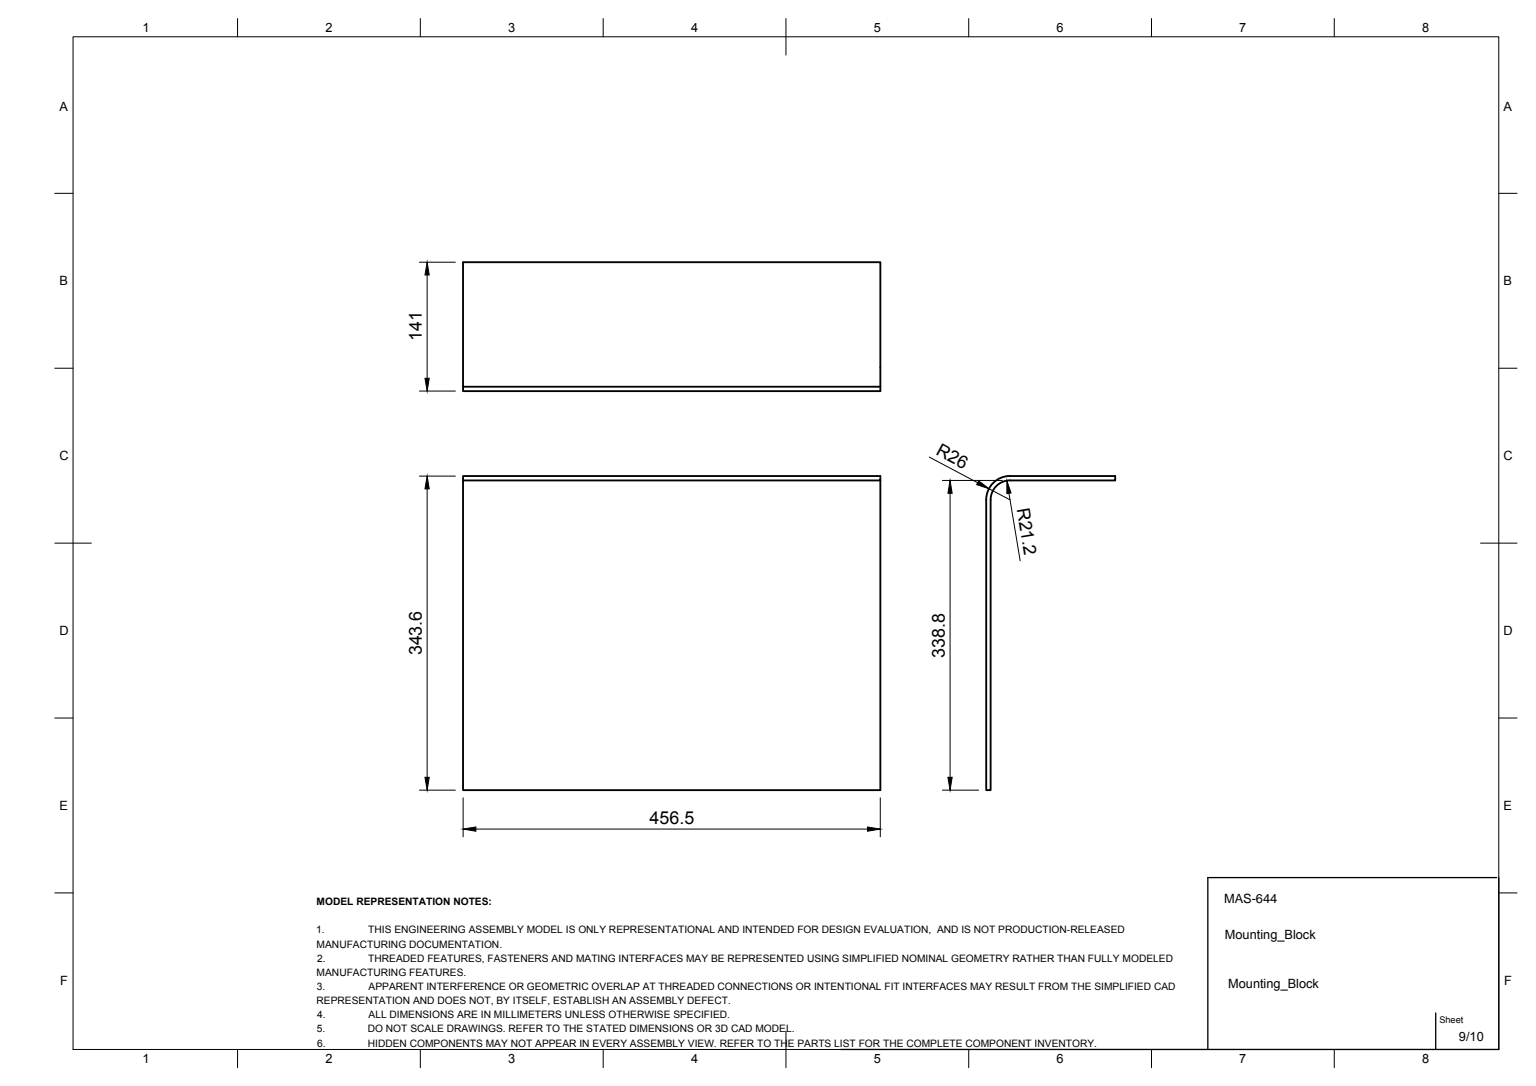
ISO-10303-21;
HEADER;
FILE_DESCRIPTION((''),'2;1');
FILE_NAME('Mounting_Block.step','2026-10-09T11:38:21-07:00',(''),(''),'','','');
FILE_SCHEMA (('AUTOMOTIVE_DESIGN { 1 0 10303 214 3 1 1 }'));
ENDSEC;
DATA;
#10=MECHANICAL_DESIGN_GEOMETRIC_PRESENTATION_REPRESENTATION('',(#65),#3619);
#49=SHAPE_REPRESENTATION_RELATIONSHIP('SRR','None',#3657,#57) ;
#57=ADVANCED_BREP_SHAPE_REPRESENTATION('',(#73),#3617) ;
#65=STYLED_ITEM('',(#3700),#73) ;
#73=MANIFOLD_SOLID_BREP('Body1',#2089) ;
#197=PLANE('',#2372) ;
#198=PLANE('',#2375) ;
#199=PLANE('',#2376) ;
#200=PLANE('',#2379) ;
#201=PLANE('',#2380) ;
#202=PLANE('',#2381) ;
#203=PLANE('',#2382) ;
#204=PLANE('',#2384) ;
#205=PLANE('',#2385) ;
#206=PLANE('',#2386) ;
#207=PLANE('',#2388) ;
#208=PLANE('',#2389) ;
#301=FACE_OUTER_BOUND('',#491,.T.) ;
#302=FACE_OUTER_BOUND('',#492,.T.) ;
#303=FACE_OUTER_BOUND('',#493,.T.) ;
#304=FACE_OUTER_BOUND('',#494,.T.) ;
#305=FACE_OUTER_BOUND('',#495,.T.) ;
#306=FACE_OUTER_BOUND('',#496,.T.) ;
#307=FACE_OUTER_BOUND('',#497,.T.) ;
#308=FACE_OUTER_BOUND('',#498,.T.) ;
#309=FACE_OUTER_BOUND('',#499,.T.) ;
#310=FACE_OUTER_BOUND('',#500,.T.) ;
#311=FACE_OUTER_BOUND('',#501,.T.) ;
#312=FACE_OUTER_BOUND('',#502,.T.) ;
#313=FACE_OUTER_BOUND('',#503,.T.) ;
#314=FACE_OUTER_BOUND('',#504,.T.) ;
#491=EDGE_LOOP('',(#1843,#1844,#1845,#1846)) ;
#492=EDGE_LOOP('',(#1847,#1848,#1849,#1850)) ;
#493=EDGE_LOOP('',(#1851,#1852,#1853,#1854)) ;
#494=EDGE_LOOP('',(#1855,#1856,#1857,#1858)) ;
#495=EDGE_LOOP('',(#1859,#1860,#1861,#1862)) ;
#496=EDGE_LOOP('',(#1863,#1864,#1865,#1866)) ;
#497=EDGE_LOOP('',(#1867,#1868,#1869,#1870)) ;
#498=EDGE_LOOP('',(#1871,#1872,#1873,#1874)) ;
#499=EDGE_LOOP('',(#1875,#1876,#1877,#1878)) ;
#500=EDGE_LOOP('',(#1879,#1880,#1881,#1882)) ;
#501=EDGE_LOOP('',(#1883,#1884,#1885,#1886)) ;
#502=EDGE_LOOP('',(#1887,#1888,#1889,#1890)) ;
#503=EDGE_LOOP('',(#1891,#1892,#1893,#1894)) ;
#504=EDGE_LOOP('',(#1895,#1896,#1897,#1898)) ;
#643=LINE('',#3510,#807) ;
#644=LINE('',#3514,#808) ;
#645=LINE('',#3518,#809) ;
#646=LINE('',#3520,#810) ;
#647=LINE('',#3521,#811) ;
#648=LINE('',#3525,#812) ;
#649=LINE('',#3529,#813) ;
#650=LINE('',#3533,#814) ;
#651=LINE('',#3535,#815) ;
#652=LINE('',#3536,#816) ;
#653=LINE('',#3539,#817) ;
#654=LINE('',#3540,#818) ;
#655=LINE('',#3541,#819) ;
#656=LINE('',#3544,#820) ;
#657=LINE('',#3545,#821) ;
#658=LINE('',#3547,#822) ;
#659=LINE('',#3548,#823) ;
#660=LINE('',#3550,#824) ;
#661=LINE('',#3553,#825) ;
#662=LINE('',#3554,#826) ;
#663=LINE('',#3557,#827) ;
#664=LINE('',#3558,#828) ;
#665=LINE('',#3560,#829) ;
#666=LINE('',#3561,#830) ;
#807=VECTOR('',#2927,1000.) ;
#808=VECTOR('',#2930,1000.) ;
#809=VECTOR('',#2935,1000.) ;
#810=VECTOR('',#2936,1000.) ;
#811=VECTOR('',#2937,1000.) ;
#812=VECTOR('',#2940,1000.) ;
#813=VECTOR('',#2943,1000.) ;
#814=VECTOR('',#2948,1000.) ;
#815=VECTOR('',#2949,1000.) ;
#816=VECTOR('',#2950,1000.) ;
#817=VECTOR('',#2953,1000.) ;
#818=VECTOR('',#2954,1000.) ;
#819=VECTOR('',#2955,1000.) ;
#820=VECTOR('',#2958,1000.) ;
#821=VECTOR('',#2959,1000.) ;
#822=VECTOR('',#2962,1000.) ;
#823=VECTOR('',#2963,1000.) ;
#824=VECTOR('',#2966,1000.) ;
#825=VECTOR('',#2969,1000.) ;
#826=VECTOR('',#2970,1000.) ;
#827=VECTOR('',#2973,1000.) ;
#828=VECTOR('',#2974,1000.) ;
#829=VECTOR('',#2977,1000.) ;
#830=VECTOR('',#2978,1000.) ;
#935=CIRCLE('',#2373,26.) ;
#936=CIRCLE('',#2374,21.2) ;
#937=CIRCLE('',#2377,26.) ;
#938=CIRCLE('',#2378,21.2) ;
#1095=VERTEX_POINT('',#3508) ;
#1096=VERTEX_POINT('',#3509) ;
#1097=VERTEX_POINT('',#3511) ;
#1098=VERTEX_POINT('',#3513) ;
#1099=VERTEX_POINT('',#3517) ;
#1100=VERTEX_POINT('',#3519) ;
#1101=VERTEX_POINT('',#3523) ;
#1102=VERTEX_POINT('',#3524) ;
#1103=VERTEX_POINT('',#3526) ;
#1104=VERTEX_POINT('',#3528) ;
#1105=VERTEX_POINT('',#3532) ;
#1106=VERTEX_POINT('',#3534) ;
#1107=VERTEX_POINT('',#3538) ;
#1108=VERTEX_POINT('',#3543) ;
#1109=VERTEX_POINT('',#3552) ;
#1110=VERTEX_POINT('',#3556) ;
#1347=EDGE_CURVE('',#1095,#1096,#643,.T.) ;
#1348=EDGE_CURVE('',#1097,#1095,#935,.T.) ;
#1349=EDGE_CURVE('',#1098,#1097,#644,.T.) ;
#1350=EDGE_CURVE('',#1098,#1096,#936,.T.) ;
#1351=EDGE_CURVE('',#1095,#1099,#645,.T.) ;
#1352=EDGE_CURVE('',#1096,#1100,#646,.T.) ;
#1353=EDGE_CURVE('',#1099,#1100,#647,.T.) ;
#1354=EDGE_CURVE('',#1101,#1102,#648,.T.) ;
#1355=EDGE_CURVE('',#1101,#1103,#937,.T.) ;
#1356=EDGE_CURVE('',#1104,#1103,#649,.T.) ;
#1357=EDGE_CURVE('',#1102,#1104,#938,.T.) ;
#1358=EDGE_CURVE('',#1105,#1101,#650,.T.) ;
#1359=EDGE_CURVE('',#1106,#1102,#651,.T.) ;
#1360=EDGE_CURVE('',#1106,#1105,#652,.T.) ;
#1361=EDGE_CURVE('',#1104,#1107,#653,.T.) ;
#1362=EDGE_CURVE('',#1100,#1107,#654,.T.) ;
#1363=EDGE_CURVE('',#1096,#1104,#655,.T.) ;
#1364=EDGE_CURVE('',#1108,#1107,#656,.T.) ;
#1365=EDGE_CURVE('',#1099,#1108,#657,.T.) ;
#1366=EDGE_CURVE('',#1103,#1108,#658,.T.) ;
#1367=EDGE_CURVE('',#1095,#1103,#659,.T.) ;
#1368=EDGE_CURVE('',#1097,#1101,#660,.T.) ;
#1369=EDGE_CURVE('',#1109,#1105,#661,.T.) ;
#1370=EDGE_CURVE('',#1109,#1097,#662,.T.) ;
#1371=EDGE_CURVE('',#1110,#1106,#663,.T.) ;
#1372=EDGE_CURVE('',#1110,#1109,#664,.T.) ;
#1373=EDGE_CURVE('',#1098,#1102,#665,.T.) ;
#1374=EDGE_CURVE('',#1110,#1098,#666,.T.) ;
#1843=ORIENTED_EDGE('',*,*,#1347,.F.) ;
#1844=ORIENTED_EDGE('',*,*,#1348,.F.) ;
#1845=ORIENTED_EDGE('',*,*,#1349,.F.) ;
#1846=ORIENTED_EDGE('',*,*,#1350,.T.) ;
#1847=ORIENTED_EDGE('',*,*,#1351,.F.) ;
#1848=ORIENTED_EDGE('',*,*,#1347,.T.) ;
#1849=ORIENTED_EDGE('',*,*,#1352,.T.) ;
#1850=ORIENTED_EDGE('',*,*,#1353,.F.) ;
#1851=ORIENTED_EDGE('',*,*,#1354,.F.) ;
#1852=ORIENTED_EDGE('',*,*,#1355,.T.) ;
#1853=ORIENTED_EDGE('',*,*,#1356,.F.) ;
#1854=ORIENTED_EDGE('',*,*,#1357,.F.) ;
#1855=ORIENTED_EDGE('',*,*,#1358,.T.) ;
#1856=ORIENTED_EDGE('',*,*,#1354,.T.) ;
#1857=ORIENTED_EDGE('',*,*,#1359,.F.) ;
#1858=ORIENTED_EDGE('',*,*,#1360,.T.) ;
#1859=ORIENTED_EDGE('',*,*,#1361,.T.) ;
#1860=ORIENTED_EDGE('',*,*,#1362,.F.) ;
#1861=ORIENTED_EDGE('',*,*,#1352,.F.) ;
#1862=ORIENTED_EDGE('',*,*,#1363,.T.) ;
#1863=ORIENTED_EDGE('',*,*,#1364,.F.) ;
#1864=ORIENTED_EDGE('',*,*,#1365,.F.) ;
#1865=ORIENTED_EDGE('',*,*,#1353,.T.) ;
#1866=ORIENTED_EDGE('',*,*,#1362,.T.) ;
#1867=ORIENTED_EDGE('',*,*,#1366,.F.) ;
#1868=ORIENTED_EDGE('',*,*,#1367,.F.) ;
#1869=ORIENTED_EDGE('',*,*,#1351,.T.) ;
#1870=ORIENTED_EDGE('',*,*,#1365,.T.) ;
#1871=ORIENTED_EDGE('',*,*,#1355,.F.) ;
#1872=ORIENTED_EDGE('',*,*,#1368,.F.) ;
#1873=ORIENTED_EDGE('',*,*,#1348,.T.) ;
#1874=ORIENTED_EDGE('',*,*,#1367,.T.) ;
#1875=ORIENTED_EDGE('',*,*,#1358,.F.) ;
#1876=ORIENTED_EDGE('',*,*,#1369,.F.) ;
#1877=ORIENTED_EDGE('',*,*,#1370,.T.) ;
#1878=ORIENTED_EDGE('',*,*,#1368,.T.) ;
#1879=ORIENTED_EDGE('',*,*,#1360,.F.) ;
#1880=ORIENTED_EDGE('',*,*,#1371,.F.) ;
#1881=ORIENTED_EDGE('',*,*,#1372,.T.) ;
#1882=ORIENTED_EDGE('',*,*,#1369,.T.) ;
#1883=ORIENTED_EDGE('',*,*,#1359,.T.) ;
#1884=ORIENTED_EDGE('',*,*,#1373,.F.) ;
#1885=ORIENTED_EDGE('',*,*,#1374,.F.) ;
#1886=ORIENTED_EDGE('',*,*,#1371,.T.) ;
#1887=ORIENTED_EDGE('',*,*,#1357,.T.) ;
#1888=ORIENTED_EDGE('',*,*,#1363,.F.) ;
#1889=ORIENTED_EDGE('',*,*,#1350,.F.) ;
#1890=ORIENTED_EDGE('',*,*,#1373,.T.) ;
#1891=ORIENTED_EDGE('',*,*,#1374,.T.) ;
#1892=ORIENTED_EDGE('',*,*,#1349,.T.) ;
#1893=ORIENTED_EDGE('',*,*,#1370,.F.) ;
#1894=ORIENTED_EDGE('',*,*,#1372,.F.) ;
#1895=ORIENTED_EDGE('',*,*,#1361,.F.) ;
#1896=ORIENTED_EDGE('',*,*,#1356,.T.) ;
#1897=ORIENTED_EDGE('',*,*,#1366,.T.) ;
#1898=ORIENTED_EDGE('',*,*,#1364,.T.) ;
#1971=CYLINDRICAL_SURFACE('',#2383,26.) ;
#1972=CYLINDRICAL_SURFACE('',#2387,21.2) ;
#2063=ADVANCED_FACE('',(#301),#197,.T.) ;
#2064=ADVANCED_FACE('',(#302),#198,.T.) ;
#2065=ADVANCED_FACE('',(#303),#199,.T.) ;
#2066=ADVANCED_FACE('',(#304),#200,.T.) ;
#2067=ADVANCED_FACE('',(#305),#201,.F.) ;
#2068=ADVANCED_FACE('',(#306),#202,.T.) ;
#2069=ADVANCED_FACE('',(#307),#203,.T.) ;
#2070=ADVANCED_FACE('',(#308),#1971,.T.) ;
#2071=ADVANCED_FACE('',(#309),#204,.T.) ;
#2072=ADVANCED_FACE('',(#310),#205,.T.) ;
#2073=ADVANCED_FACE('',(#311),#206,.F.) ;
#2074=ADVANCED_FACE('',(#312),#1972,.F.) ;
#2075=ADVANCED_FACE('',(#313),#207,.F.) ;
#2076=ADVANCED_FACE('',(#314),#208,.T.) ;
#2089=CLOSED_SHELL('',(#2063,#2064,#2065,#2066,#2067,#2068,#2069,#2070,
#2071,#2072,#2073,#2074,#2075,#2076)) ;
#2371=AXIS2_PLACEMENT_3D('',#3506,#2923,#2924) ;
#2372=AXIS2_PLACEMENT_3D('',#3507,#2925,#2926) ;
#2373=AXIS2_PLACEMENT_3D('',#3512,#2928,#2929) ;
#2374=AXIS2_PLACEMENT_3D('',#3515,#2931,#2932) ;
#2375=AXIS2_PLACEMENT_3D('',#3516,#2933,#2934) ;
#2376=AXIS2_PLACEMENT_3D('',#3522,#2938,#2939) ;
#2377=AXIS2_PLACEMENT_3D('',#3527,#2941,#2942) ;
#2378=AXIS2_PLACEMENT_3D('',#3530,#2944,#2945) ;
#2379=AXIS2_PLACEMENT_3D('',#3531,#2946,#2947) ;
#2380=AXIS2_PLACEMENT_3D('',#3537,#2951,#2952) ;
#2381=AXIS2_PLACEMENT_3D('',#3542,#2956,#2957) ;
#2382=AXIS2_PLACEMENT_3D('',#3546,#2960,#2961) ;
#2383=AXIS2_PLACEMENT_3D('',#3549,#2964,#2965) ;
#2384=AXIS2_PLACEMENT_3D('',#3551,#2967,#2968) ;
#2385=AXIS2_PLACEMENT_3D('',#3555,#2971,#2972) ;
#2386=AXIS2_PLACEMENT_3D('',#3559,#2975,#2976) ;
#2387=AXIS2_PLACEMENT_3D('',#3562,#2979,#2980) ;
#2388=AXIS2_PLACEMENT_3D('',#3563,#2981,#2982) ;
#2389=AXIS2_PLACEMENT_3D('',#3564,#2983,#2984) ;
#2923=DIRECTION('axis',(0.,0.,1.)) ;
#2924=DIRECTION('refdir',(1.,0.,0.)) ;
#2925=DIRECTION('center_axis',(0.,0.,1.)) ;
#2926=DIRECTION('ref_axis',(1.,0.,0.)) ;
#2927=DIRECTION('',(0.,1.,0.)) ;
#2928=DIRECTION('center_axis',(0.,0.,-1.)) ;
#2929=DIRECTION('ref_axis',(-1.,0.,0.)) ;
#2930=DIRECTION('',(1.,7.2280144832367E-15,0.)) ;
#2931=DIRECTION('center_axis',(0.,0.,-1.)) ;
#2932=DIRECTION('ref_axis',(1.,0.,0.)) ;
#2933=DIRECTION('center_axis',(0.,0.,1.)) ;
#2934=DIRECTION('ref_axis',(1.,0.,0.)) ;
#2935=DIRECTION('',(-1.,-1.22464679914735E-16,0.)) ;
#2936=DIRECTION('',(-1.,-1.22464679914735E-16,0.)) ;
#2937=DIRECTION('',(0.,1.,0.)) ;
#2938=DIRECTION('center_axis',(0.,0.,-1.)) ;
#2939=DIRECTION('ref_axis',(-1.,0.,0.)) ;
#2940=DIRECTION('',(-1.,-7.2280144832367E-15,0.)) ;
#2941=DIRECTION('center_axis',(0.,0.,-1.)) ;
#2942=DIRECTION('ref_axis',(-1.,0.,0.)) ;
#2943=DIRECTION('',(0.,-1.,0.)) ;
#2944=DIRECTION('center_axis',(0.,0.,-1.)) ;
#2945=DIRECTION('ref_axis',(1.,0.,0.)) ;
#2946=DIRECTION('center_axis',(0.,0.,-1.)) ;
#2947=DIRECTION('ref_axis',(-1.,0.,0.)) ;
#2948=DIRECTION('',(0.,-1.,0.)) ;
#2949=DIRECTION('',(0.,-1.,0.)) ;
#2950=DIRECTION('',(1.,0.,0.)) ;
#2951=DIRECTION('center_axis',(1.22464679914735E-16,-1.,0.)) ;
#2952=DIRECTION('ref_axis',(1.,1.22464679914735E-16,0.)) ;
#2953=DIRECTION('',(-1.,-1.22464679914735E-16,0.)) ;
#2954=DIRECTION('',(0.,0.,-1.)) ;
#2955=DIRECTION('',(0.,0.,-1.)) ;
#2956=DIRECTION('center_axis',(-1.,0.,0.)) ;
#2957=DIRECTION('ref_axis',(0.,0.,1.)) ;
#2958=DIRECTION('',(0.,1.,0.)) ;
#2959=DIRECTION('',(0.,0.,-1.)) ;
#2960=DIRECTION('center_axis',(1.22464679914735E-16,-1.,0.)) ;
#2961=DIRECTION('ref_axis',(1.,1.22464679914735E-16,0.)) ;
#2962=DIRECTION('',(-1.,-1.22464679914735E-16,0.)) ;
#2963=DIRECTION('',(0.,0.,-1.)) ;
#2964=DIRECTION('center_axis',(0.,0.,-1.)) ;
#2965=DIRECTION('ref_axis',(-1.,0.,0.)) ;
#2966=DIRECTION('',(0.,0.,-1.)) ;
#2967=DIRECTION('center_axis',(1.,0.,0.)) ;
#2968=DIRECTION('ref_axis',(0.,0.,-1.)) ;
#2969=DIRECTION('',(0.,0.,-1.)) ;
#2970=DIRECTION('',(0.,-1.,0.)) ;
#2971=DIRECTION('center_axis',(0.,1.,0.)) ;
#2972=DIRECTION('ref_axis',(0.,0.,1.)) ;
#2973=DIRECTION('',(0.,0.,-1.)) ;
#2974=DIRECTION('',(1.,0.,0.)) ;
#2975=DIRECTION('center_axis',(1.,0.,0.)) ;
#2976=DIRECTION('ref_axis',(0.,0.,-1.)) ;
#2977=DIRECTION('',(0.,0.,-1.)) ;
#2978=DIRECTION('',(0.,-1.,0.)) ;
#2979=DIRECTION('center_axis',(0.,0.,-1.)) ;
#2980=DIRECTION('ref_axis',(-1.,0.,0.)) ;
#2981=DIRECTION('center_axis',(0.,0.,-1.)) ;
#2982=DIRECTION('ref_axis',(-1.,0.,0.)) ;
#2983=DIRECTION('center_axis',(0.,0.,-1.)) ;
#2984=DIRECTION('ref_axis',(-1.,0.,0.)) ;
#3506=CARTESIAN_POINT('',(0.,0.,0.)) ;
#3507=CARTESIAN_POINT('Origin',(294.2,409.,456.5)) ;
#3508=CARTESIAN_POINT('',(294.2,409.,456.5)) ;
#3509=CARTESIAN_POINT('',(294.2,413.8,456.5)) ;
#3510=CARTESIAN_POINT('',(294.2,409.,456.5)) ;
#3511=CARTESIAN_POINT('',(320.2,435.000000000001,456.5)) ;
#3512=CARTESIAN_POINT('Origin',(294.2,435.,456.5)) ;
#3513=CARTESIAN_POINT('',(315.4,435.,456.5)) ;
#3514=CARTESIAN_POINT('',(315.4,435.,456.5)) ;
#3515=CARTESIAN_POINT('Origin',(294.2,435.,456.5)) ;
#3516=CARTESIAN_POINT('Origin',(315.4,435.,456.5)) ;
#3517=CARTESIAN_POINT('',(-23.4000000000002,409.,456.5)) ;
#3518=CARTESIAN_POINT('',(294.2,409.,456.5)) ;
#3519=CARTESIAN_POINT('',(-23.4000000000002,413.8,456.5)) ;
#3520=CARTESIAN_POINT('',(294.2,413.8,456.5)) ;
#3521=CARTESIAN_POINT('',(-23.4000000000002,409.,456.5)) ;
#3522=CARTESIAN_POINT('Origin',(320.2,435.000000000001,-5.55111512312578E-14)) ;
#3523=CARTESIAN_POINT('',(320.2,435.000000000001,-5.55111512312578E-14)) ;
#3524=CARTESIAN_POINT('',(315.4,435.,-5.55111512312578E-14)) ;
#3525=CARTESIAN_POINT('',(320.2,435.000000000001,-5.55111512312578E-14)) ;
#3526=CARTESIAN_POINT('',(294.2,409.,-5.55111512312578E-14)) ;
#3527=CARTESIAN_POINT('Origin',(294.2,435.,-5.55111512312578E-14)) ;
#3528=CARTESIAN_POINT('',(294.2,413.8,-5.55111512312578E-14)) ;
#3529=CARTESIAN_POINT('',(294.2,413.8,-5.55111512312578E-14)) ;
#3530=CARTESIAN_POINT('Origin',(294.2,435.,-5.55111512312578E-14)) ;
#3531=CARTESIAN_POINT('Origin',(294.2,413.8,-5.55111512312578E-14)) ;
#3532=CARTESIAN_POINT('',(320.2,550.,-5.55111512312578E-14)) ;
#3533=CARTESIAN_POINT('',(320.2,550.,-5.55111512312578E-14)) ;
#3534=CARTESIAN_POINT('',(315.4,550.,-5.55111512312578E-14)) ;
#3535=CARTESIAN_POINT('',(315.4,550.,-5.55111512312578E-14)) ;
#3536=CARTESIAN_POINT('',(315.4,550.,-5.55111512312578E-14)) ;
#3537=CARTESIAN_POINT('Origin',(294.2,413.8,456.5)) ;
#3538=CARTESIAN_POINT('',(-23.4000000000002,413.8,-5.55111512312578E-14)) ;
#3539=CARTESIAN_POINT('',(294.2,413.8,-5.55111512312578E-14)) ;
#3540=CARTESIAN_POINT('',(-23.4000000000002,413.8,456.5)) ;
#3541=CARTESIAN_POINT('',(294.2,413.8,456.5)) ;
#3542=CARTESIAN_POINT('Origin',(-23.4000000000002,409.,456.5)) ;
#3543=CARTESIAN_POINT('',(-23.4000000000002,409.,-5.55111512312578E-14)) ;
#3544=CARTESIAN_POINT('',(-23.4000000000002,409.,-5.55111512312578E-14)) ;
#3545=CARTESIAN_POINT('',(-23.4000000000002,409.,456.5)) ;
#3546=CARTESIAN_POINT('Origin',(294.2,409.,456.5)) ;
#3547=CARTESIAN_POINT('',(294.2,409.,-5.55111512312578E-14)) ;
#3548=CARTESIAN_POINT('',(294.2,409.,456.5)) ;
#3549=CARTESIAN_POINT('Origin',(294.2,435.,456.5)) ;
#3550=CARTESIAN_POINT('',(320.2,435.000000000001,456.5)) ;
#3551=CARTESIAN_POINT('Origin',(320.2,550.,456.5)) ;
#3552=CARTESIAN_POINT('',(320.2,550.,456.5)) ;
#3553=CARTESIAN_POINT('',(320.2,550.,456.5)) ;
#3554=CARTESIAN_POINT('',(320.2,550.,456.5)) ;
#3555=CARTESIAN_POINT('Origin',(315.4,550.,456.5)) ;
#3556=CARTESIAN_POINT('',(315.4,550.,456.5)) ;
#3557=CARTESIAN_POINT('',(315.4,550.,456.5)) ;
#3558=CARTESIAN_POINT('',(315.4,550.,456.5)) ;
#3559=CARTESIAN_POINT('Origin',(315.4,550.,456.5)) ;
#3560=CARTESIAN_POINT('',(315.4,435.,456.5)) ;
#3561=CARTESIAN_POINT('',(315.4,550.,456.5)) ;
#3562=CARTESIAN_POINT('Origin',(294.2,435.,456.5)) ;
#3563=CARTESIAN_POINT('Origin',(294.2,435.,456.5)) ;
#3564=CARTESIAN_POINT('Origin',(294.2,435.,-5.55111512312578E-14)) ;
#3607=UNCERTAINTY_MEASURE_WITH_UNIT(LENGTH_MEASURE(0.01),#3620,
'DISTANCE_ACCURACY_VALUE',
'Maximum model space distance between geometric entities at asserted c
onnectivities') ;
#3609=UNCERTAINTY_MEASURE_WITH_UNIT(LENGTH_MEASURE(0.01),#3620,
'DISTANCE_ACCURACY_VALUE',
'Maximum model space distance between geometric entities at asserted c
onnectivities') ;
#3617=(
GEOMETRIC_REPRESENTATION_CONTEXT(3)
GLOBAL_UNCERTAINTY_ASSIGNED_CONTEXT((#3607))
GLOBAL_UNIT_ASSIGNED_CONTEXT((#3620,#3622,#3623))
REPRESENTATION_CONTEXT('','3D')
) ;
#3619=(
GEOMETRIC_REPRESENTATION_CONTEXT(3)
GLOBAL_UNCERTAINTY_ASSIGNED_CONTEXT((#3609))
GLOBAL_UNIT_ASSIGNED_CONTEXT((#3620,#3622,#3623))
REPRESENTATION_CONTEXT('','3D')
) ;
#3620=(
LENGTH_UNIT()
NAMED_UNIT(*)
SI_UNIT(.MILLI.,.METRE.)
) ;
#3622=(
NAMED_UNIT(*)
PLANE_ANGLE_UNIT()
SI_UNIT($,.RADIAN.)
) ;
#3623=(
NAMED_UNIT(*)
SI_UNIT($,.STERADIAN.)
SOLID_ANGLE_UNIT()
) ;
#3631=SHAPE_DEFINITION_REPRESENTATION(#3640,#3657) ;
#3640=PRODUCT_DEFINITION_SHAPE('',$,#3667) ;
#3657=SHAPE_REPRESENTATION('',(#2371),#3617) ;
#3659=PRODUCT_DEFINITION_CONTEXT('part definition',#3688,'design') ;
#3667=PRODUCT_DEFINITION('Mounting_Block','Mounting_Block',#3676,#3659) ;
#3676=PRODUCT_DEFINITION_FORMATION('',$,#3697) ;
#3688=APPLICATION_CONTEXT(
'Core Data for Automotive Mechanical Design Process') ;
#3689=PRODUCT_CONTEXT('part definition',#3688,'mechanical') ;
#3697=PRODUCT('Mounting_Block','Mounting_Block',$,(#3689)) ;
#3700=PRESENTATION_STYLE_ASSIGNMENT((#3702)) ;
#3702=SURFACE_STYLE_USAGE(.BOTH.,#3704) ;
#3704=SURFACE_SIDE_STYLE('',(#3706)) ;
#3706=SURFACE_STYLE_FILL_AREA(#3708) ;
#3708=FILL_AREA_STYLE('Opaque(202,209,238)',(#3710)) ;
#3710=FILL_AREA_STYLE_COLOUR('Opaque(202,209,238)',#3712) ;
#3712=COLOUR_RGB('Opaque(202,209,238)', 0.09019608, 0.27058824, 0.51372549) ;
ENDSEC;
END-ISO-10303-21;
